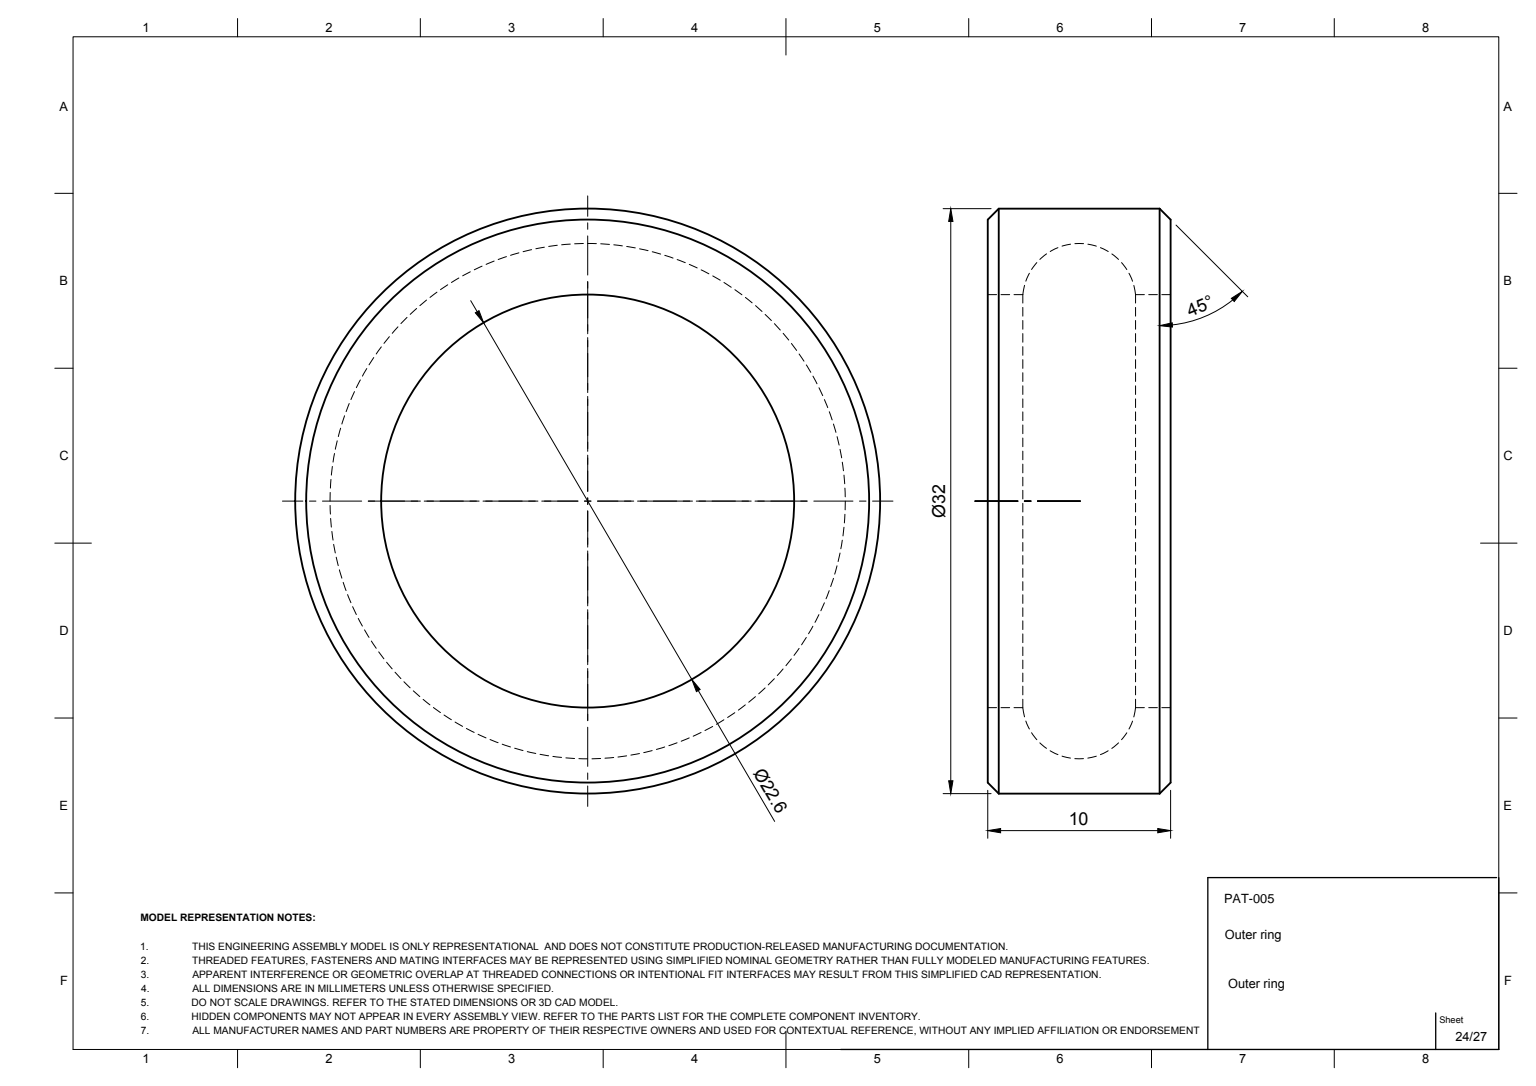
ISO-10303-21;
HEADER;
/* Generated by software containing ST-Developer
 * from STEP Tools, Inc. (www.steptools.com) 
 */

FILE_DESCRIPTION(
/* description */ ('Ball-race swivel caster'),
/* implementation_level */ '2;1');

FILE_NAME(
/* name */ 'Outer ring.step',
/* time_stamp */ '2026-10-29T16:15:51-07:00',
/* author */ (''),
/* organization */ (''),
/* preprocessor_version */ 'ST-DEVELOPER v20.2',
/* originating_system */ 'Autodesk Translation Framework v15.17.0.0',
/* authorisation */ '');

FILE_SCHEMA (('AUTOMOTIVE_DESIGN { 1 0 10303 214 3 1 1 }'));
ENDSEC;

DATA;
#10=MECHANICAL_DESIGN_GEOMETRIC_PRESENTATION_REPRESENTATION('',(#322),#7816);
#32=CONICAL_SURFACE('',#4377,1.57,0.785398163397449);
#33=CONICAL_SURFACE('',#4381,1.57,0.785398163397449);
#191=TOROIDAL_SURFACE('',#4366,1.1,0.309556);
#273=SHAPE_REPRESENTATION_RELATIONSHIP('SRR','None',#7922,#293);
#293=ADVANCED_BREP_SHAPE_REPRESENTATION('',(#357),#7811);
#322=STYLED_ITEM('',(#8097),#357);
#357=MANIFOLD_SOLID_BREP('Body1',#3729);
#429=FACE_BOUND('',#961,.T.);
#430=FACE_BOUND('',#966,.T.);
#508=PLANE('',#4374);
#509=PLANE('',#4383);
#689=FACE_OUTER_BOUND('',#958,.T.);
#690=FACE_OUTER_BOUND('',#959,.T.);
#691=FACE_OUTER_BOUND('',#960,.T.);
#692=FACE_OUTER_BOUND('',#962,.T.);
#693=FACE_OUTER_BOUND('',#963,.T.);
#694=FACE_OUTER_BOUND('',#964,.T.);
#695=FACE_OUTER_BOUND('',#965,.T.);
#696=FACE_OUTER_BOUND('',#967,.T.);
#958=EDGE_LOOP('',(#3249,#3250,#3251,#3252,#3253,#3254));
#959=EDGE_LOOP('',(#3255,#3256,#3257,#3258,#3259));
#960=EDGE_LOOP('',(#3260));
#961=EDGE_LOOP('',(#3261));
#962=EDGE_LOOP('',(#3262,#3263,#3264,#3265));
#963=EDGE_LOOP('',(#3266,#3267,#3268,#3269));
#964=EDGE_LOOP('',(#3270,#3271,#3272,#3273));
#965=EDGE_LOOP('',(#3274));
#966=EDGE_LOOP('',(#3275));
#967=EDGE_LOOP('',(#3276,#3277,#3278,#3279,#3280));
#1153=LINE('',#7264,#1308);
#1154=LINE('',#7273,#1309);
#1155=LINE('',#7277,#1310);
#1156=LINE('',#7281,#1311);
#1157=LINE('',#7284,#1312);
#1308=VECTOR('',#5455,1.129765);
#1309=VECTOR('',#5466,1.57);
#1310=VECTOR('',#5471,1.6);
#1311=VECTOR('',#5476,1.57);
#1312=VECTOR('',#5481,1.129765);
#1523=CIRCLE('',#4367,1.129765);
#1524=CIRCLE('',#4368,1.129765);
#1525=CIRCLE('',#4369,0.309556);
#1526=CIRCLE('',#4370,1.129765);
#1527=CIRCLE('',#4371,1.129765);
#1528=CIRCLE('',#4373,1.129765);
#1529=CIRCLE('',#4375,1.54);
#1530=CIRCLE('',#4376,1.129765);
#1531=CIRCLE('',#4378,1.6);
#1532=CIRCLE('',#4380,1.6);
#1533=CIRCLE('',#4382,1.54);
#1868=VERTEX_POINT('',#7252);
#1869=VERTEX_POINT('',#7253);
#1870=VERTEX_POINT('',#7256);
#1871=VERTEX_POINT('',#7258);
#1872=VERTEX_POINT('',#7262);
#1873=VERTEX_POINT('',#7266);
#1874=VERTEX_POINT('',#7268);
#1875=VERTEX_POINT('',#7271);
#1876=VERTEX_POINT('',#7275);
#1877=VERTEX_POINT('',#7279);
#2344=EDGE_CURVE('',#1868,#1869,#1523,.T.);
#2345=EDGE_CURVE('',#1869,#1868,#1524,.T.);
#2346=EDGE_CURVE('',#1869,#1870,#1525,.T.);
#2347=EDGE_CURVE('',#1871,#1870,#1526,.T.);
#2348=EDGE_CURVE('',#1870,#1871,#1527,.T.);
#2349=EDGE_CURVE('',#1872,#1872,#1528,.T.);
#2350=EDGE_CURVE('',#1872,#1871,#1153,.T.);
#2351=EDGE_CURVE('',#1873,#1873,#1529,.T.);
#2352=EDGE_CURVE('',#1874,#1874,#1530,.T.);
#2353=EDGE_CURVE('',#1875,#1875,#1531,.T.);
#2354=EDGE_CURVE('',#1875,#1873,#1154,.T.);
#2355=EDGE_CURVE('',#1876,#1876,#1532,.T.);
#2356=EDGE_CURVE('',#1876,#1875,#1155,.T.);
#2357=EDGE_CURVE('',#1877,#1877,#1533,.T.);
#2358=EDGE_CURVE('',#1877,#1876,#1156,.T.);
#2359=EDGE_CURVE('',#1868,#1874,#1157,.T.);
#3249=ORIENTED_EDGE('',*,*,#2344,.F.);
#3250=ORIENTED_EDGE('',*,*,#2345,.F.);
#3251=ORIENTED_EDGE('',*,*,#2346,.T.);
#3252=ORIENTED_EDGE('',*,*,#2347,.F.);
#3253=ORIENTED_EDGE('',*,*,#2348,.F.);
#3254=ORIENTED_EDGE('',*,*,#2346,.F.);
#3255=ORIENTED_EDGE('',*,*,#2349,.T.);
#3256=ORIENTED_EDGE('',*,*,#2350,.T.);
#3257=ORIENTED_EDGE('',*,*,#2347,.T.);
#3258=ORIENTED_EDGE('',*,*,#2348,.T.);
#3259=ORIENTED_EDGE('',*,*,#2350,.F.);
#3260=ORIENTED_EDGE('',*,*,#2351,.F.);
#3261=ORIENTED_EDGE('',*,*,#2352,.T.);
#3262=ORIENTED_EDGE('',*,*,#2353,.F.);
#3263=ORIENTED_EDGE('',*,*,#2354,.T.);
#3264=ORIENTED_EDGE('',*,*,#2351,.T.);
#3265=ORIENTED_EDGE('',*,*,#2354,.F.);
#3266=ORIENTED_EDGE('',*,*,#2355,.F.);
#3267=ORIENTED_EDGE('',*,*,#2356,.T.);
#3268=ORIENTED_EDGE('',*,*,#2353,.T.);
#3269=ORIENTED_EDGE('',*,*,#2356,.F.);
#3270=ORIENTED_EDGE('',*,*,#2357,.F.);
#3271=ORIENTED_EDGE('',*,*,#2358,.T.);
#3272=ORIENTED_EDGE('',*,*,#2355,.T.);
#3273=ORIENTED_EDGE('',*,*,#2358,.F.);
#3274=ORIENTED_EDGE('',*,*,#2357,.T.);
#3275=ORIENTED_EDGE('',*,*,#2349,.F.);
#3276=ORIENTED_EDGE('',*,*,#2344,.T.);
#3277=ORIENTED_EDGE('',*,*,#2345,.T.);
#3278=ORIENTED_EDGE('',*,*,#2359,.T.);
#3279=ORIENTED_EDGE('',*,*,#2352,.F.);
#3280=ORIENTED_EDGE('',*,*,#2359,.F.);
#3484=CYLINDRICAL_SURFACE('',#4372,1.129765);
#3485=CYLINDRICAL_SURFACE('',#4379,1.6);
#3486=CYLINDRICAL_SURFACE('',#4384,1.129765);
#3660=ADVANCED_FACE('',(#689),#191,.F.);
#3661=ADVANCED_FACE('',(#690),#3484,.F.);
#3662=ADVANCED_FACE('',(#691,#429),#508,.T.);
#3663=ADVANCED_FACE('',(#692),#32,.T.);
#3664=ADVANCED_FACE('',(#693),#3485,.T.);
#3665=ADVANCED_FACE('',(#694),#33,.T.);
#3666=ADVANCED_FACE('',(#695,#430),#509,.T.);
#3667=ADVANCED_FACE('',(#696),#3486,.F.);
#3729=CLOSED_SHELL('',(#3660,#3661,#3662,#3663,#3664,#3665,#3666,#3667));
#4365=AXIS2_PLACEMENT_3D('',#7250,#5437,#5438);
#4366=AXIS2_PLACEMENT_3D('',#7251,#5439,#5440);
#4367=AXIS2_PLACEMENT_3D('',#7254,#5441,#5442);
#4368=AXIS2_PLACEMENT_3D('',#7255,#5443,#5444);
#4369=AXIS2_PLACEMENT_3D('',#7257,#5445,#5446);
#4370=AXIS2_PLACEMENT_3D('',#7259,#5447,#5448);
#4371=AXIS2_PLACEMENT_3D('',#7260,#5449,#5450);
#4372=AXIS2_PLACEMENT_3D('',#7261,#5451,#5452);
#4373=AXIS2_PLACEMENT_3D('',#7263,#5453,#5454);
#4374=AXIS2_PLACEMENT_3D('',#7265,#5456,#5457);
#4375=AXIS2_PLACEMENT_3D('',#7267,#5458,#5459);
#4376=AXIS2_PLACEMENT_3D('',#7269,#5460,#5461);
#4377=AXIS2_PLACEMENT_3D('',#7270,#5462,#5463);
#4378=AXIS2_PLACEMENT_3D('',#7272,#5464,#5465);
#4379=AXIS2_PLACEMENT_3D('',#7274,#5467,#5468);
#4380=AXIS2_PLACEMENT_3D('',#7276,#5469,#5470);
#4381=AXIS2_PLACEMENT_3D('',#7278,#5472,#5473);
#4382=AXIS2_PLACEMENT_3D('',#7280,#5474,#5475);
#4383=AXIS2_PLACEMENT_3D('',#7282,#5477,#5478);
#4384=AXIS2_PLACEMENT_3D('',#7283,#5479,#5480);
#5437=DIRECTION('axis',(0.,0.,1.));
#5438=DIRECTION('refdir',(1.,0.,0.));
#5439=DIRECTION('center_axis',(0.,-1.,0.));
#5440=DIRECTION('ref_axis',(0.,0.,-1.));
#5441=DIRECTION('center_axis',(0.,-1.,0.));
#5442=DIRECTION('ref_axis',(1.,0.,0.));
#5443=DIRECTION('center_axis',(0.,-1.,0.));
#5444=DIRECTION('ref_axis',(1.,0.,0.));
#5445=DIRECTION('center_axis',(1.,0.,1.22464679914735E-16));
#5446=DIRECTION('ref_axis',(-1.22464679914735E-16,0.,1.));
#5447=DIRECTION('center_axis',(0.,1.,0.));
#5448=DIRECTION('ref_axis',(1.,0.,0.));
#5449=DIRECTION('center_axis',(0.,1.,0.));
#5450=DIRECTION('ref_axis',(1.,0.,0.));
#5451=DIRECTION('center_axis',(0.,-1.,0.));
#5452=DIRECTION('ref_axis',(1.,0.,0.));
#5453=DIRECTION('center_axis',(0.,-1.,0.));
#5454=DIRECTION('ref_axis',(1.,0.,0.));
#5455=DIRECTION('',(0.,1.,0.));
#5456=DIRECTION('center_axis',(0.,1.,0.));
#5457=DIRECTION('ref_axis',(0.,0.,1.));
#5458=DIRECTION('center_axis',(0.,-1.,0.));
#5459=DIRECTION('ref_axis',(1.,0.,0.));
#5460=DIRECTION('center_axis',(0.,-1.,0.));
#5461=DIRECTION('ref_axis',(1.,0.,0.));
#5462=DIRECTION('center_axis',(0.,-1.,0.));
#5463=DIRECTION('ref_axis',(1.,0.,0.));
#5464=DIRECTION('center_axis',(0.,-1.,0.));
#5465=DIRECTION('ref_axis',(1.,0.,0.));
#5466=DIRECTION('',(0.707106781186548,0.707106781186547,8.65956056235494E-17));
#5467=DIRECTION('center_axis',(0.,-1.,0.));
#5468=DIRECTION('ref_axis',(1.,0.,0.));
#5469=DIRECTION('center_axis',(0.,-1.,0.));
#5470=DIRECTION('ref_axis',(1.,0.,0.));
#5471=DIRECTION('',(0.,1.,0.));
#5472=DIRECTION('center_axis',(0.,1.,0.));
#5473=DIRECTION('ref_axis',(1.,0.,0.));
#5474=DIRECTION('center_axis',(0.,-1.,0.));
#5475=DIRECTION('ref_axis',(1.,0.,0.));
#5476=DIRECTION('',(-0.707106781186548,0.707106781186547,-8.65956056235494E-17));
#5477=DIRECTION('center_axis',(0.,-1.,0.));
#5478=DIRECTION('ref_axis',(0.,0.,-1.));
#5479=DIRECTION('center_axis',(0.,-1.,0.));
#5480=DIRECTION('ref_axis',(1.,0.,0.));
#5481=DIRECTION('',(0.,1.,0.));
#7250=CARTESIAN_POINT('',(0.,0.,0.));
#7251=CARTESIAN_POINT('Origin',(0.,0.,0.));
#7252=CARTESIAN_POINT('',(-1.129765,0.308121667383195,-1.38356309103871E-16));
#7253=CARTESIAN_POINT('',(-1.38356309103871E-16,0.308121667383195,1.129765));
#7254=CARTESIAN_POINT('Origin',(0.,0.308121667383195,0.));
#7255=CARTESIAN_POINT('Origin',(0.,0.308121667383195,0.));
#7256=CARTESIAN_POINT('',(-1.38356309103871E-16,-0.308121667383195,1.129765));
#7257=CARTESIAN_POINT('Origin',(-1.34711147906209E-16,0.,1.1));
#7258=CARTESIAN_POINT('',(-1.129765,-0.308121667383195,1.38356309103871E-16));
#7259=CARTESIAN_POINT('Origin',(0.,-0.308121667383195,0.));
#7260=CARTESIAN_POINT('Origin',(0.,-0.308121667383195,0.));
#7261=CARTESIAN_POINT('Origin',(0.,0.,0.));
#7262=CARTESIAN_POINT('',(-1.129765,-0.5,-1.38356309103871E-16));
#7263=CARTESIAN_POINT('Origin',(0.,-0.5,0.));
#7264=CARTESIAN_POINT('',(-1.129765,0.,-1.38356309103871E-16));
#7265=CARTESIAN_POINT('Origin',(1.54,0.5,0.));
#7266=CARTESIAN_POINT('',(-1.54,0.5,-1.88595607068692E-16));
#7267=CARTESIAN_POINT('Origin',(0.,0.5,0.));
#7268=CARTESIAN_POINT('',(-1.129765,0.5,-1.38356309103871E-16));
#7269=CARTESIAN_POINT('Origin',(0.,0.5,0.));
#7270=CARTESIAN_POINT('Origin',(0.,0.47,0.));
#7271=CARTESIAN_POINT('',(-1.6,0.44,-1.95943487863577E-16));
#7272=CARTESIAN_POINT('Origin',(0.,0.44,0.));
#7273=CARTESIAN_POINT('',(-1.57,0.47,-1.92269547466134E-16));
#7274=CARTESIAN_POINT('Origin',(0.,0.,0.));
#7275=CARTESIAN_POINT('',(-1.6,-0.44,-1.95943487863577E-16));
#7276=CARTESIAN_POINT('Origin',(0.,-0.44,0.));
#7277=CARTESIAN_POINT('',(-1.6,0.,-1.95943487863577E-16));
#7278=CARTESIAN_POINT('Origin',(0.,-0.47,0.));
#7279=CARTESIAN_POINT('',(-1.54,-0.5,-1.88595607068692E-16));
#7280=CARTESIAN_POINT('Origin',(0.,-0.5,0.));
#7281=CARTESIAN_POINT('',(-1.57,-0.47,-1.92269547466134E-16));
#7282=CARTESIAN_POINT('Origin',(1.129765,-0.5,0.));
#7283=CARTESIAN_POINT('Origin',(0.,0.,0.));
#7284=CARTESIAN_POINT('',(-1.129765,0.,-1.38356309103871E-16));
#7784=UNCERTAINTY_MEASURE_WITH_UNIT(LENGTH_MEASURE(0.001),#7817,
'DISTANCE_ACCURACY_VALUE',
'Maximum model space distance between geometric entities at asserted c
onnectivities');
#7789=UNCERTAINTY_MEASURE_WITH_UNIT(LENGTH_MEASURE(0.001),#7817,
'DISTANCE_ACCURACY_VALUE',
'Maximum model space distance between geometric entities at asserted c
onnectivities');
#7811=(
GEOMETRIC_REPRESENTATION_CONTEXT(3)
GLOBAL_UNCERTAINTY_ASSIGNED_CONTEXT((#7784))
GLOBAL_UNIT_ASSIGNED_CONTEXT((#7817,#7819,#7820))
REPRESENTATION_CONTEXT('','3D')
);
#7816=(
GEOMETRIC_REPRESENTATION_CONTEXT(3)
GLOBAL_UNCERTAINTY_ASSIGNED_CONTEXT((#7789))
GLOBAL_UNIT_ASSIGNED_CONTEXT((#7817,#7819,#7820))
REPRESENTATION_CONTEXT('','3D')
);
#7817=(
LENGTH_UNIT()
NAMED_UNIT(*)
SI_UNIT(.CENTI.,.METRE.)
);
#7819=(
NAMED_UNIT(*)
PLANE_ANGLE_UNIT()
SI_UNIT($,.RADIAN.)
);
#7820=(
NAMED_UNIT(*)
SI_UNIT($,.STERADIAN.)
SOLID_ANGLE_UNIT()
);
#7842=SHAPE_DEFINITION_REPRESENTATION(#7883,#7922);
#7883=PRODUCT_DEFINITION_SHAPE('',$,#7949);
#7922=SHAPE_REPRESENTATION('',(#4365),#7811);
#7927=PRODUCT_DEFINITION_CONTEXT('part definition',#8007,'design');
#7949=PRODUCT_DEFINITION('Outer ring','Outer ring',#7975,#7927);
#7975=PRODUCT_DEFINITION_FORMATION('',$,#8030);
#8007=APPLICATION_CONTEXT(
'Core Data for Automotive Mechanical Design Process');
#8008=PRODUCT_CONTEXT('part definition',#8007,'mechanical');
#8030=PRODUCT('Outer ring','Outer ring','Outer ring',(#8008));
#8091=COLOUR_RGB('Grey',0.48,0.52,0.57);
#8092=FILL_AREA_STYLE_COLOUR('',#8091);
#8093=FILL_AREA_STYLE('',(#8092));
#8094=SURFACE_STYLE_FILL_AREA(#8093);
#8095=SURFACE_SIDE_STYLE('',(#8094));
#8096=SURFACE_STYLE_USAGE(.BOTH.,#8095);
#8097=PRESENTATION_STYLE_ASSIGNMENT((#8096));
ENDSEC;
END-ISO-10303-21;
